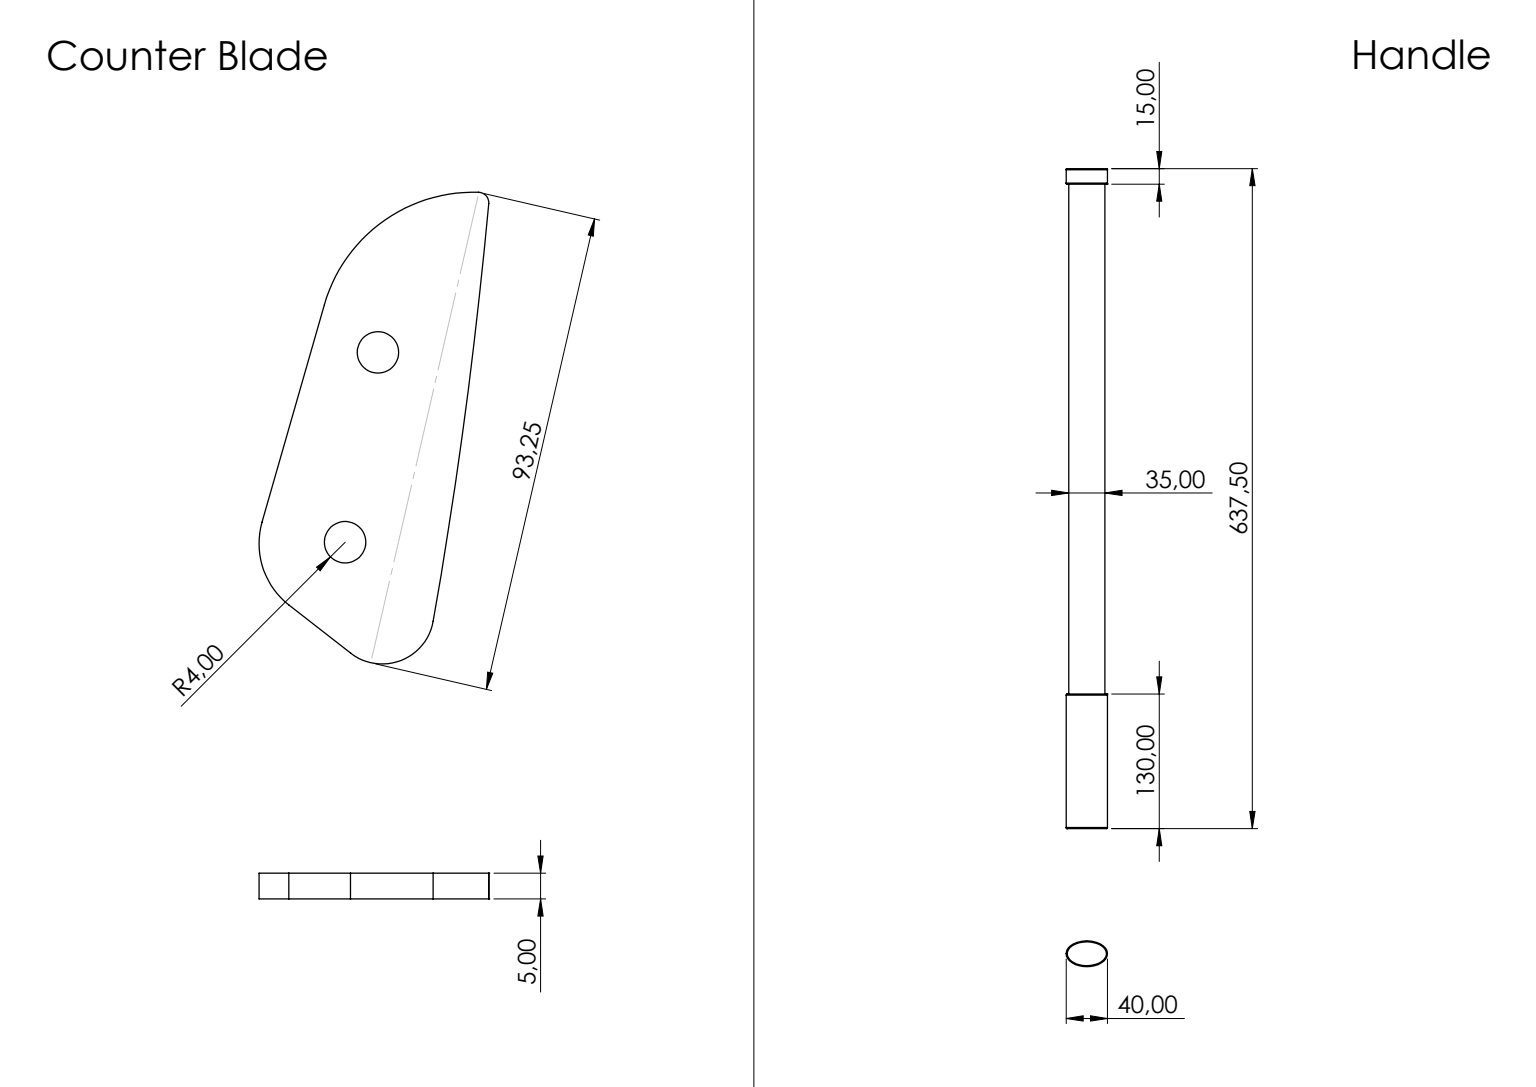
ISO-10303-21;
HEADER;
FILE_DESCRIPTION (('STEP AP214'),
    '1' );
FILE_NAME ('Counter Blade.step',
    '2026-10-06T08:24:18',
    ( '' ),
    ( '' ),
    'SwSTEP 2.0',
    'SolidWorks 2020',
    '' );
FILE_SCHEMA (( 'AUTOMOTIVE_DESIGN' ));
ENDSEC;

DATA;
#10=ORIENTED_EDGE ( 'NONE', *, *, #9690, .T. ) ;
#46=SHAPE_REPRESENTATION_RELATIONSHIP ( 'NONE' , 'NONE' ,  #1832, #4657 ) ;
#47=ADVANCED_FACE ( 'NONE', ( #10008 ), #1731, .T. ) ;
#57=AXIS2_PLACEMENT_3D ( 'NONE', #266, #1824, #2572 ) ;
#90=CARTESIAN_POINT ( 'NONE',  ( -6.594989095229207621, -2.500000000000000000, -526.5005977704149700 ) ) ;
#108=ORIENTED_EDGE ( 'NONE', *, *, #6819, .T. ) ;
#128=UNCERTAINTY_MEASURE_WITH_UNIT (LENGTH_MEASURE( 1.000000000000000082E-05 ), #4984, 'distance_accuracy_value', 'NONE');
#150=DIRECTION ( 'NONE',  ( 0.000000000000000000, 1.000000000000000000, -0.000000000000000000 ) ) ;
#154=LINE ( 'NONE', #4186, #6919 ) ;
#194=DIRECTION ( 'NONE',  ( 0.000000000000000000, 1.000000000000000000, -0.000000000000000000 ) ) ;
#199=VERTEX_POINT ( 'NONE', #5447 ) ;
#218=AXIS2_PLACEMENT_3D ( 'NONE', #4647, #8943, #6415 ) ;
#229=AXIS2_PLACEMENT_3D ( 'NONE', #4133, #4730, #3920 ) ;
#252=FACE_OUTER_BOUND ( 'NONE', #958, .T. ) ;
#266=CARTESIAN_POINT ( 'NONE',  ( -28.01838671672410896, -7.500000000000000000, -497.7560445212019999 ) ) ;
#274=CARTESIAN_POINT ( 'NONE',  ( -24.05731444175778577, -2.500000000000000000, -497.1993521173619683 ) ) ;
#286=PRODUCT_DEFINITION ( 'UNKNOWN', '', #449, #10550 ) ;
#328=FILL_AREA_STYLE_COLOUR ( '', #2300 ) ;
#356=EDGE_LOOP ( 'NONE', ( #3781, #10603 ) ) ;
#358=CYLINDRICAL_SURFACE ( 'NONE', #9948, 4.000000000000000000 ) ;
#380=DIRECTION ( 'NONE',  ( -0.9612616959383296633, 0.000000000000000000, -0.2756373558169616933 ) ) ;
#449=PRODUCT_DEFINITION_FORMATION_WITH_SPECIFIED_SOURCE ( 'ANY', '', #8602, .NOT_KNOWN. ) ;
#467=PRODUCT_DEFINITION_SHAPE ( 'NONE', 'NONE',  #286 ) ;
#471=VERTEX_POINT ( 'NONE', #3146 ) ;
#479=CARTESIAN_POINT ( 'NONE',  ( -30.41084982323499730, -2.500000000000000000, -460.5301199443746327 ) ) ;
#492=CARTESIAN_POINT ( 'NONE',  ( -36.01445213885307339, -7.500000000000000000, -460.8005622778243264 ) ) ;
#498=PLANE ( 'NONE',  #1895 ) ;
#557=AXIS2_PLACEMENT_3D ( 'NONE', #8920, #6558, #7364 ) ;
#585=DIRECTION ( 'NONE',  ( 0.000000000000000000, 1.000000000000000000, -0.000000000000000000 ) ) ;
#595=AXIS2_PLACEMENT_3D ( 'NONE', #9903, #3452, #2538 ) ;
#688=EDGE_LOOP ( 'NONE', ( #10453, #7051, #5685, #108 ) ) ;
#691=CARTESIAN_POINT ( 'NONE',  ( -1002.398135702230206, -7.500000000000000000, -618.0215964952759577 ) ) ;
#726=VERTEX_POINT ( 'NONE', #7376 ) ;
#745=DIRECTION ( 'NONE',  ( 0.000000000000000000, 1.000000000000000000, -0.000000000000000000 ) ) ;
#772=UNCERTAINTY_MEASURE_WITH_UNIT (LENGTH_MEASURE( 1.000000000000000082E-05 ), #971, 'distance_accuracy_value', 'NONE');
#788=ORIENTED_EDGE ( 'NONE', *, *, #10618, .F. ) ;
#791=ORIENTED_EDGE ( 'NONE', *, *, #4315, .T. ) ;
#819=ADVANCED_FACE ( 'NONE', ( #8387 ), #3450, .T. ) ;
#898=FILL_AREA_STYLE_COLOUR ( '', #2976 ) ;
#926=VECTOR ( 'NONE', #7594, 1000.000000000000227 ) ;
#927=ORIENTED_EDGE ( 'NONE', *, *, #1491, .T. ) ;
#933=CIRCLE ( 'NONE', #9689, 10.00000000000000178 ) ;
#958=EDGE_LOOP ( 'NONE', ( #5843, #3891, #8722, #3360 ) ) ;
#964=ADVANCED_FACE ( 'NONE', ( #9287 ), #358, .F. ) ;
#971=( LENGTH_UNIT ( ) NAMED_UNIT ( * ) SI_UNIT ( .MILLI., .METRE. ) );
#1064=ORIENTED_EDGE ( 'NONE', *, *, #5099, .F. ) ;
#1076=CIRCLE ( 'NONE', #229, 10.00000000000001599 ) ;
#1082=UNCERTAINTY_MEASURE_WITH_UNIT (LENGTH_MEASURE( 1.000000000000000082E-05 ), #1763, 'distance_accuracy_value', 'NONE');
#1091=CARTESIAN_POINT ( 'NONE',  ( -9.542482902900836450, -2.500000000000000000, -498.6999609700373526 ) ) ;
#1094=ADVANCED_FACE ( 'NONE', ( #9274 ), #5124, .T. ) ;
#1098=CIRCLE ( 'NONE', #1446, 4.000000000000000000 ) ;
#1129=PRESENTATION_STYLE_ASSIGNMENT (( #3395 ) ) ;
#1155=EDGE_LOOP ( 'NONE', ( #7696, #1064, #1796, #10507 ) ) ;
#1171=CARTESIAN_POINT ( 'NONE',  ( -38.33299437316763658, -7.500000000000000000, -461.6435047520546391 ) ) ;
#1209=DIRECTION ( 'NONE',  ( 0.000000000000000000, 1.000000000000000000, -0.000000000000000000 ) ) ;
#1225=DIRECTION ( 'NONE',  ( 0.000000000000000000, 1.000000000000000000, -0.000000000000000000 ) ) ;
#1279=DIRECTION ( 'NONE',  ( 0.000000000000000000, 1.000000000000000000, -0.000000000000000000 ) ) ;
#1282=AXIS2_PLACEMENT_3D ( 'NONE', #5388, #3631, #4388 ) ;
#1287=ADVANCED_FACE ( 'NONE', ( #1841, #7740, #3559 ), #8492, .T. ) ;
#1294=CARTESIAN_POINT ( 'NONE',  ( -50.43337757792475173, -7.500000000000000000, -464.9351226150769207 ) ) ;
#1402=DIRECTION ( 'NONE',  ( 0.000000000000000000, -1.000000000000000000, -0.000000000000000000 ) ) ;
#1416=VERTEX_POINT ( 'NONE', #7205 ) ;
#1428=DIRECTION ( 'NONE',  ( 0.000000000000000000, -1.000000000000000000, 0.000000000000000000 ) ) ;
#1446=AXIS2_PLACEMENT_3D ( 'NONE', #2951, #3606, #3652 ) ;
#1463=DIRECTION ( 'NONE',  ( 0.000000000000000000, 1.000000000000000000, -0.000000000000000000 ) ) ;
#1491=EDGE_CURVE ( 'NONE', #3141, #3262, #1508, .T. ) ;
#1492=FACE_OUTER_BOUND ( 'NONE', #688, .T. ) ;
#1508=LINE ( 'NONE', #8502, #7111 ) ;
#1544=DIRECTION ( 'NONE',  ( 0.9902680687415800209, 0.000000000000000000, 0.1391731009599966873 ) ) ;
#1552=( NAMED_UNIT ( * ) PLANE_ANGLE_UNIT ( ) SI_UNIT ( $, .RADIAN. ) );
#1553=EDGE_CURVE ( 'NONE', #471, #9652, #10117, .T. ) ;
#1577=EDGE_CURVE ( 'NONE', #3224, #9652, #4271, .T. ) ;
#1588=ORIENTED_EDGE ( 'NONE', *, *, #1491, .F. ) ;
#1602=CIRCLE ( 'NONE', #8454, 29.99999999999998224 ) ;
#1620=FACE_OUTER_BOUND ( 'NONE', #6632, .T. ) ;
#1669=CYLINDRICAL_SURFACE ( 'NONE', #557, 2.000000000000003997 ) ;
#1680=EDGE_LOOP ( 'NONE', ( #8671, #5541, #1588, #1899 ) ) ;
#1731=PLANE ( 'NONE',  #595 ) ;
#1763=( LENGTH_UNIT ( ) NAMED_UNIT ( * ) SI_UNIT ( .MILLI., .METRE. ) );
#1773=ORIENTED_EDGE ( 'NONE', *, *, #3982, .F. ) ;
#1781=CARTESIAN_POINT ( 'NONE',  ( -50.43337757792475173, -2.500000000000000000, -464.9351226150769207 ) ) ;
#1796=ORIENTED_EDGE ( 'NONE', *, *, #9999, .T. ) ;
#1824=DIRECTION ( 'NONE',  ( 0.000000000000000000, 1.000000000000000000, -0.000000000000000000 ) ) ;
#1832=SHAPE_REPRESENTATION ( 'Counter Blade', ( #2817 ), #5369 ) ;
#1841=FACE_BOUND ( 'NONE', #5066, .T. ) ;
#1889=SURFACE_SIDE_STYLE ('',( #10003 ) ) ;
#1895=AXIS2_PLACEMENT_3D ( 'NONE', #7059, #1402, #2107 ) ;
#1899=ORIENTED_EDGE ( 'NONE', *, *, #7170, .T. ) ;
#1905=ORIENTED_EDGE ( 'NONE', *, *, #4115, .F. ) ;
#1958=DIRECTION ( 'NONE',  ( -0.9902680687415801319, 0.000000000000000000, -0.1391731009599957991 ) ) ;
#1967=CARTESIAN_POINT ( 'NONE',  ( -38.33299437316763658, -7.500000000000000000, -461.6435047520546391 ) ) ;
#1999=DIRECTION ( 'NONE',  ( 0.000000000000000000, -1.000000000000000000, -0.000000000000000000 ) ) ;
#2026=CIRCLE ( 'NONE', #9059, 15.00000000000000533 ) ;
#2034=ORIENTED_EDGE ( 'NONE', *, *, #1553, .F. ) ;
#2039=CARTESIAN_POINT ( 'NONE',  ( -31.97945899169042505, -7.500000000000000000, -498.3127369250419747 ) ) ;
#2048=EDGE_CURVE ( 'NONE', #3465, #199, #5327, .T. ) ;
#2051=CARTESIAN_POINT ( 'NONE',  ( -38.38033378105252780, -7.500000000000000000, -506.9690816445435644 ) ) ;
#2055=CARTESIAN_POINT ( 'NONE',  ( -8.586595388443328147, -7.500000000000000000, -526.6836397678595176 ) ) ;
#2065=DIRECTION ( 'NONE',  ( 0.000000000000000000, -1.000000000000000000, 0.000000000000000000 ) ) ;
#2107=DIRECTION ( 'NONE',  ( -0.9902680687415799099, 0.000000000000000000, -0.1391731009599969648 ) ) ;
#2116=CARTESIAN_POINT ( 'NONE',  ( -38.38033378105252780, -2.500000000000000000, -506.9690816445435644 ) ) ;
#2145=CARTESIAN_POINT ( 'NONE',  ( -8.518317708839887814, -7.500000000000000000, -528.6824739677025491 ) ) ;
#2214=DIRECTION ( 'NONE',  ( 0.9902680687415800209, 0.000000000000000000, 0.1391731009599966873 ) ) ;
#2245=DIRECTION ( 'NONE',  ( 0.9958031466069998672, 0.000000000000000000, 0.09152099872487109988 ) ) ;
#2264=EDGE_CURVE ( 'NONE', #3224, #3141, #2026, .T. ) ;
#2266=LINE ( 'NONE', #5533, #6349 ) ;
#2291=VECTOR ( 'NONE', #585, 1000.000000000000000 ) ;
#2300=COLOUR_RGB ( '', 0.09019608, 0.27058824, 0.51372549) ;
#2318=DIRECTION ( 'NONE',  ( 0.000000000000000000, 1.000000000000000000, -0.000000000000000000 ) ) ;
#2325=ORIENTED_EDGE ( 'NONE', *, *, #2474, .F. ) ;
#2336=ORIENTED_EDGE ( 'NONE', *, *, #1553, .T. ) ;
#2372=LINE ( 'NONE', #7314, #10423 ) ;
#2373=CARTESIAN_POINT ( 'NONE',  ( -34.37192209820132405, -7.500000000000000000, -461.0868123482146643 ) ) ;
#2408=CARTESIAN_POINT ( 'NONE',  ( -50.43337757792475173, -7.500000000000000000, -464.9351226150769207 ) ) ;
#2409=AXIS2_PLACEMENT_3D ( 'NONE', #10577, #745, #5681 ) ;
#2445=FACE_OUTER_BOUND ( 'NONE', #1155, .T. ) ;
#2446=ORIENTED_EDGE ( 'NONE', *, *, #3484, .T. ) ;
#2457=VECTOR ( 'NONE', #2065, 1000.000000000000000 ) ;
#2474=EDGE_CURVE ( 'NONE', #7593, #3224, #2372, .T. ) ;
#2495=CARTESIAN_POINT ( 'NONE',  ( -34.37192209820132405, -7.500000000000000000, -461.0868123482146643 ) ) ;
#2511=DIRECTION ( 'NONE',  ( 0.000000000000000000, 1.000000000000000000, -0.000000000000000000 ) ) ;
#2538=DIRECTION ( 'NONE',  ( 0.000000000000000000, 1.000000000000000000, -0.000000000000000000 ) ) ;
#2550=CYLINDRICAL_SURFACE ( 'NONE', #7930, 10.00000000000001599 ) ;
#2572=DIRECTION ( 'NONE',  ( -0.9902680687415800209, 0.000000000000000000, -0.1391731009599967983 ) ) ;
#2623=DIRECTION ( 'NONE',  ( 0.9902680687415800209, 0.000000000000000000, 0.1391731009599966873 ) ) ;
#2659=ORIENTED_EDGE ( 'NONE', *, *, #6694, .F. ) ;
#2661=EDGE_LOOP ( 'NONE', ( #3907, #10072, #9299, #3463 ) ) ;
#2702=CARTESIAN_POINT ( 'NONE',  ( -19.08872200864999868, -7.500000000000000000, -429.3350920981999934 ) ) ;
#2709=DIRECTION ( 'NONE',  ( 0.03413883980201725538, 0.000000000000000000, -0.9994170999222358187 ) ) ;
#2757=CIRCLE ( 'NONE', #6859, 999.9999999999997726 ) ;
#2758=CARTESIAN_POINT ( 'NONE',  ( -33.34106825788445150, -2.500000000000000000, -439.6766126514281154 ) ) ;
#2767=FACE_BOUND ( 'NONE', #4216, .T. ) ;
#2817=AXIS2_PLACEMENT_3D ( 'NONE', #8634, #3966, #3161 ) ;
#2835=CIRCLE ( 'NONE', #1282, 29.99999999999998224 ) ;
#2951=CARTESIAN_POINT ( 'NONE',  ( -28.01838671672410896, -7.500000000000000000, -497.7560445212019999 ) ) ;
#2976=COLOUR_RGB ( '', 0.09019608, 0.27058824, 0.51372549) ;
#2997=AXIS2_PLACEMENT_3D ( 'NONE', #7933, #9712, #1544 ) ;
#3058=ORIENTED_EDGE ( 'NONE', *, *, #7135, .T. ) ;
#3127=ORIENTED_EDGE ( 'NONE', *, *, #6034, .T. ) ;
#3131=EDGE_LOOP ( 'NONE', ( #791, #3679 ) ) ;
#3138=DIRECTION ( 'NONE',  ( -0.9612616959383299964, 0.000000000000000000, -0.2756373558169601945 ) ) ;
#3141=VERTEX_POINT ( 'NONE', #1294 ) ;
#3142=FACE_OUTER_BOUND ( 'NONE', #9330, .T. ) ;
#3146=CARTESIAN_POINT ( 'NONE',  ( -33.34106825788445150, -2.500000000000000000, -439.6766126514281154 ) ) ;
#3150=CIRCLE ( 'NONE', #9164, 14.99999999999999112 ) ;
#3157=CARTESIAN_POINT ( 'NONE',  ( -8.518317708839887814, -2.500000000000000000, -528.6824739677025491 ) ) ;
#3158=CARTESIAN_POINT ( 'NONE',  ( -8.586595388443328147, -2.500000000000000000, -526.6836397678595176 ) ) ;
#3161=DIRECTION ( 'NONE',  ( 1.000000000000000000, 0.000000000000000000, 0.000000000000000000 ) ) ;
#3209=EDGE_LOOP ( 'NONE', ( #3058, #3445, #4855, #6669, #927, #4767, #7906 ) ) ;
#3224=VERTEX_POINT ( 'NONE', #7055 ) ;
#3228=FACE_OUTER_BOUND ( 'NONE', #3258, .T. ) ;
#3258=EDGE_LOOP ( 'NONE', ( #5813, #4124, #3127, #7270 ) ) ;
#3262=VERTEX_POINT ( 'NONE', #2051 ) ;
#3329=ORIENTED_EDGE ( 'NONE', *, *, #8250, .F. ) ;
#3351=ADVANCED_FACE ( 'NONE', ( #3228 ), #8062, .F. ) ;
#3360=ORIENTED_EDGE ( 'NONE', *, *, #8250, .T. ) ;
#3379=ADVANCED_FACE ( 'NONE', ( #1620 ), #1669, .T. ) ;
#3395=SURFACE_STYLE_USAGE ( .BOTH. , #1889 ) ;
#3424=CARTESIAN_POINT ( 'NONE',  ( -34.37192209820132405, -7.500000000000000000, -461.0868123482146643 ) ) ;
#3439=AXIS2_PLACEMENT_3D ( 'NONE', #7852, #10078, #2214 ) ;
#3445=ORIENTED_EDGE ( 'NONE', *, *, #5099, .T. ) ;
#3450=PLANE ( 'NONE',  #5140 ) ;
#3452=DIRECTION ( 'NONE',  ( -0.6156614753245244209, 0.000000000000000000, 0.7880107536076078611 ) ) ;
#3463=ORIENTED_EDGE ( 'NONE', *, *, #10535, .F. ) ;
#3464=DIRECTION ( 'NONE',  ( 0.000000000000000000, 1.000000000000000000, -0.000000000000000000 ) ) ;
#3465=VERTEX_POINT ( 'NONE', #2039 ) ;
#3484=EDGE_CURVE ( 'NONE', #7857, #199, #8968, .T. ) ;
#3505=CARTESIAN_POINT ( 'NONE',  ( -53.22217373880035041, -2.500000000000000000, -455.2094346026838139 ) ) ;
#3529=ORIENTED_EDGE ( 'NONE', *, *, #8365, .F. ) ;
#3546=EDGE_LOOP ( 'NONE', ( #1905, #1773, #10, #788 ) ) ;
#3559=FACE_OUTER_BOUND ( 'NONE', #3209, .T. ) ;
#3606=DIRECTION ( 'NONE',  ( 0.000000000000000000, 1.000000000000000000, -0.000000000000000000 ) ) ;
#3626=CARTESIAN_POINT ( 'NONE',  ( -36.01445213885307339, -7.656480000000000175, -460.8005622778243264 ) ) ;
#3631=DIRECTION ( 'NONE',  ( 0.000000000000000000, -1.000000000000000000, 0.000000000000000000 ) ) ;
#3636=CARTESIAN_POINT ( 'NONE',  ( -28.01838671672410896, -7.500000000000000000, -497.7560445212019999 ) ) ;
#3641=VECTOR ( 'NONE', #4192, 1000.000000000000227 ) ;
#3652=DIRECTION ( 'NONE',  ( 0.9902680687415800209, 0.000000000000000000, 0.1391731009599966873 ) ) ;
#3679=ORIENTED_EDGE ( 'NONE', *, *, #8962, .T. ) ;
#3710=EDGE_CURVE ( 'NONE', #7593, #471, #154, .T. ) ;
#3768=DIRECTION ( 'NONE',  ( 0.000000000000000000, 1.000000000000000000, -0.000000000000000000 ) ) ;
#3781=ORIENTED_EDGE ( 'NONE', *, *, #6819, .F. ) ;
#3881=CYLINDRICAL_SURFACE ( 'NONE', #3439, 4.000000000000000000 ) ;
#3891=ORIENTED_EDGE ( 'NONE', *, *, #7244, .F. ) ;
#3907=ORIENTED_EDGE ( 'NONE', *, *, #7170, .F. ) ;
#3920=DIRECTION ( 'NONE',  ( -0.6156614753245235327, 0.000000000000000000, 0.7880107536076085273 ) ) ;
#3944=CARTESIAN_POINT ( 'NONE',  ( -9.542482902900836450, -7.500000000000000000, -498.6999609700373526 ) ) ;
#3966=DIRECTION ( 'NONE',  ( 0.000000000000000000, 0.000000000000000000, 1.000000000000000000 ) ) ;
#3976=VECTOR ( 'NONE', #5351, 1000.000000000000000 ) ;
#3982=EDGE_CURVE ( 'NONE', #9423, #3262, #8509, .T. ) ;
#4038=SHAPE_DEFINITION_REPRESENTATION ( #467, #1832 ) ;
#4076=( NAMED_UNIT ( * ) SI_UNIT ( $, .STERADIAN. ) SOLID_ANGLE_UNIT ( ) );
#4115=EDGE_CURVE ( 'NONE', #3262, #7113, #1602, .T. ) ;
#4124=ORIENTED_EDGE ( 'NONE', *, *, #7586, .F. ) ;
#4130=AXIS2_PLACEMENT_3D ( 'NONE', #8785, #1428, #4714 ) ;
#4133=CARTESIAN_POINT ( 'NONE',  ( -27.18445350464674348, -2.500000000000000000, -447.5567201875090291 ) ) ;
#4186=CARTESIAN_POINT ( 'NONE',  ( -33.34106825788445150, -7.500000000000000000, -439.6766126514281154 ) ) ;
#4192=DIRECTION ( 'NONE',  ( 0.2756373558169616378, 0.000000000000000000, -0.9612616959383295523 ) ) ;
#4216=EDGE_LOOP ( 'NONE', ( #2659, #3329 ) ) ;
#4221=LINE ( 'NONE', #8295, #5908 ) ;
#4257=( NAMED_UNIT ( * ) PLANE_ANGLE_UNIT ( ) SI_UNIT ( $, .RADIAN. ) );
#4259=EDGE_CURVE ( 'NONE', #471, #6686, #1076, .T. ) ;
#4271=LINE ( 'NONE', #7541, #8819 ) ;
#4303=AXIS2_PLACEMENT_3D ( 'NONE', #3158, #8905, #8793 ) ;
#4315=EDGE_CURVE ( 'NONE', #3465, #8821, #8795, .T. ) ;
#4388=DIRECTION ( 'NONE',  ( -0.9612616959383299964, 0.000000000000000000, -0.2756373558169601945 ) ) ;
#4440=DIRECTION ( 'NONE',  ( 0.9902680687415800209, 0.000000000000000000, 0.1391731009599966873 ) ) ;
#4499=DIRECTION ( 'NONE',  ( -0.9902680687415800209, 0.000000000000000000, -0.1391731009599967983 ) ) ;
#4647=CARTESIAN_POINT ( 'NONE',  ( -1002.398135702230206, -2.500000000000000000, -618.0215964952759577 ) ) ;
#4657=ADVANCED_BREP_SHAPE_REPRESENTATION ( '', ( #8917, #2817 ), #5369 ) ;
#4694=ADVANCED_FACE ( 'NONE', ( #9005 ), #6691, .T. ) ;
#4714=DIRECTION ( 'NONE',  ( 0.9958031466069998672, 0.000000000000000000, 0.09152099872487109988 ) ) ;
#4727=LINE ( 'NONE', #2145, #2291 ) ;
#4730=DIRECTION ( 'NONE',  ( 0.000000000000000000, 1.000000000000000000, -0.000000000000000000 ) ) ;
#4767=ORIENTED_EDGE ( 'NONE', *, *, #4115, .T. ) ;
#4791=EDGE_CURVE ( 'NONE', #8821, #7857, #4221, .T. ) ;
#4845=CARTESIAN_POINT ( 'NONE',  ( -24.05731444175778577, -7.500000000000000000, -497.1993521173619683 ) ) ;
#4855=ORIENTED_EDGE ( 'NONE', *, *, #2474, .T. ) ;
#4882=( NAMED_UNIT ( * ) PLANE_ANGLE_UNIT ( ) SI_UNIT ( $, .RADIAN. ) );
#4984=( LENGTH_UNIT ( ) NAMED_UNIT ( * ) SI_UNIT ( .MILLI., .METRE. ) );
#5032=MECHANICAL_DESIGN_GEOMETRIC_PRESENTATION_REPRESENTATION('',(#5209),#7957);
#5066=EDGE_LOOP ( 'NONE', ( #8248, #8698 ) ) ;
#5078=LINE ( 'NONE', #5944, #9694 ) ;
#5094=ORIENTED_EDGE ( 'NONE', *, *, #7000, .T. ) ;
#5099=EDGE_CURVE ( 'NONE', #1416, #7593, #933, .T. ) ;
#5124=CYLINDRICAL_SURFACE ( 'NONE', #6944, 29.99999999999999289 ) ;
#5140=AXIS2_PLACEMENT_3D ( 'NONE', #3505, #380, #8335 ) ;
#5209=STYLED_ITEM ( 'NONE', ( #8160 ), #4657 ) ;
#5235=ORIENTED_EDGE ( 'NONE', *, *, #7135, .F. ) ;
#5241=ORIENTED_EDGE ( 'NONE', *, *, #4259, .T. ) ;
#5255=SURFACE_SIDE_STYLE ('',( #8316 ) ) ;
#5306=CARTESIAN_POINT ( 'NONE',  ( -28.01838671672410896, -2.500000000000000000, -497.7560445212019999 ) ) ;
#5327=LINE ( 'NONE', #6190, #7681 ) ;
#5350=VERTEX_POINT ( 'NONE', #1967 ) ;
#5351=DIRECTION ( 'NONE',  ( 0.000000000000000000, 1.000000000000000000, -0.000000000000000000 ) ) ;
#5369=( GEOMETRIC_REPRESENTATION_CONTEXT ( 3 ) GLOBAL_UNCERTAINTY_ASSIGNED_CONTEXT ( ( #128 ) ) GLOBAL_UNIT_ASSIGNED_CONTEXT ( ( #4984, #4882, #5733 ) ) REPRESENTATION_CONTEXT ( 'NONE', 'WORKASPACE' ) );
#5382=CLOSED_SHELL ( 'NONE', ( #3351, #8609, #9379, #964, #1287, #6194, #6341, #47, #4694, #819, #1094, #3379, #8631 ) ) ;
#5388=CARTESIAN_POINT ( 'NONE',  ( -9.542482902900836450, -2.500000000000000000, -498.6999609700373526 ) ) ;
#5422=DIRECTION ( 'NONE',  ( -0.6156614753245245319, 0.000000000000000000, 0.7880107536076076391 ) ) ;
#5423=AXIS2_PLACEMENT_3D ( 'NONE', #2702, #1999, #7533 ) ;
#5447=CARTESIAN_POINT ( 'NONE',  ( -31.97945899169042505, -2.500000000000000000, -498.3127369250419747 ) ) ;
#5457=LINE ( 'NONE', #1171, #3976 ) ;
#5463=CARTESIAN_POINT ( 'NONE',  ( -36.01445213885307339, -2.500000000000000000, -460.8005622778243264 ) ) ;
#5533=CARTESIAN_POINT ( 'NONE',  ( -30.41084982323499730, -7.500000000000000000, -460.5301199443746327 ) ) ;
#5541=ORIENTED_EDGE ( 'NONE', *, *, #3982, .T. ) ;
#5579=CARTESIAN_POINT ( 'NONE',  ( -38.33299437316763658, -2.500000000000000000, -461.6435047520546391 ) ) ;
#5648=AXIS2_PLACEMENT_3D ( 'NONE', #3424, #150, #2623 ) ;
#5681=DIRECTION ( 'NONE',  ( 0.9902680687415800209, 0.000000000000000000, 0.1391731009599966873 ) ) ;
#5685=ORIENTED_EDGE ( 'NONE', *, *, #2048, .T. ) ;
#5733=( NAMED_UNIT ( * ) SI_UNIT ( $, .STERADIAN. ) SOLID_ANGLE_UNIT ( ) );
#5741=CIRCLE ( 'NONE', #6247, 2.000000000000007550 ) ;
#5765=ORIENTED_EDGE ( 'NONE', *, *, #7000, .F. ) ;
#5813=ORIENTED_EDGE ( 'NONE', *, *, #8719, .F. ) ;
#5823=CIRCLE ( 'NONE', #4130, 999.9999999999997726 ) ;
#5837=FILL_AREA_STYLE ('',( #898 ) ) ;
#5843=ORIENTED_EDGE ( 'NONE', *, *, #6034, .F. ) ;
#5900=EDGE_CURVE ( 'NONE', #8899, #9423, #9938, .T. ) ;
#5908=VECTOR ( 'NONE', #194, 1000.000000000000000 ) ;
#5944=CARTESIAN_POINT ( 'NONE',  ( -6.594989095229207621, -7.500000000000000000, -526.5005977704149700 ) ) ;
#6034=EDGE_CURVE ( 'NONE', #5350, #9268, #5457, .T. ) ;
#6049=AXIS2_PLACEMENT_3D ( 'NONE', #5306, #1225, #9452 ) ;
#6098=ORIENTED_EDGE ( 'NONE', *, *, #2048, .F. ) ;
#6190=CARTESIAN_POINT ( 'NONE',  ( -31.97945899169042505, -7.500000000000000000, -498.3127369250419747 ) ) ;
#6194=ADVANCED_FACE ( 'NONE', ( #3142 ), #8837, .T. ) ;
#6247=AXIS2_PLACEMENT_3D ( 'NONE', #2055, #8595, #2709 ) ;
#6268=ORIENTED_EDGE ( 'NONE', *, *, #9945, .F. ) ;
#6341=ADVANCED_FACE ( 'NONE', ( #2445 ), #2550, .T. ) ;
#6349=VECTOR ( 'NONE', #1463, 1000.000000000000000 ) ;
#6370=ORIENTED_EDGE ( 'NONE', *, *, #9690, .F. ) ;
#6415=DIRECTION ( 'NONE',  ( -0.9902680687415799099, 0.000000000000000000, -0.1391731009599970204 ) ) ;
#6433=DIRECTION ( 'NONE',  ( 0.000000000000000000, 1.000000000000000000, -0.000000000000000000 ) ) ;
#6441=DIRECTION ( 'NONE',  ( 0.000000000000000000, -1.000000000000000000, 0.000000000000000000 ) ) ;
#6451=PRODUCT_CONTEXT ( 'NONE', #9844, 'mechanical' ) ;
#6516=CIRCLE ( 'NONE', #9431, 4.000000000000003553 ) ;
#6525=ORIENTED_EDGE ( 'NONE', *, *, #5900, .F. ) ;
#6539=CYLINDRICAL_SURFACE ( 'NONE', #2997, 4.000000000000000000 ) ;
#6558=DIRECTION ( 'NONE',  ( 0.000000000000000000, 1.000000000000000000, -0.000000000000000000 ) ) ;
#6624=CARTESIAN_POINT ( 'NONE',  ( -17.33381025012258903, -2.500000000000000000, -445.8348527500487535 ) ) ;
#6632=EDGE_LOOP ( 'NONE', ( #8804, #6268, #7935, #5765 ) ) ;
#6669=ORIENTED_EDGE ( 'NONE', *, *, #2264, .T. ) ;
#6686=VERTEX_POINT ( 'NONE', #6624 ) ;
#6691=CYLINDRICAL_SURFACE ( 'NONE', #8313, 14.99999999999999112 ) ;
#6694=EDGE_CURVE ( 'NONE', #9268, #10547, #9289, .T. ) ;
#6744=DIRECTION ( 'NONE',  ( 0.2756373558169616378, 0.000000000000000000, -0.9612616959383295523 ) ) ;
#6783=ORIENTED_EDGE ( 'NONE', *, *, #8962, .F. ) ;
#6819=EDGE_CURVE ( 'NONE', #199, #7857, #8932, .T. ) ;
#6859=AXIS2_PLACEMENT_3D ( 'NONE', #691, #8961, #2245 ) ;
#6908=DIRECTION ( 'NONE',  ( 0.000000000000000000, 1.000000000000000000, -0.000000000000000000 ) ) ;
#6919=VECTOR ( 'NONE', #8470, 1000.000000000000000 ) ;
#6944=AXIS2_PLACEMENT_3D ( 'NONE', #1091, #10073, #1958 ) ;
#6947=MECHANICAL_DESIGN_GEOMETRIC_PRESENTATION_REPRESENTATION('',(#8299),#9675);
#7000=EDGE_CURVE ( 'NONE', #8559, #10046, #7895, .T. ) ;
#7019=ORIENTED_EDGE ( 'NONE', *, *, #1577, .F. ) ;
#7037=CIRCLE ( 'NONE', #5648, 4.000000000000000000 ) ;
#7051=ORIENTED_EDGE ( 'NONE', *, *, #4315, .F. ) ;
#7055=CARTESIAN_POINT ( 'NONE',  ( -45.24937426871918689, -7.500000000000000000, -448.9804009737068213 ) ) ;
#7059=CARTESIAN_POINT ( 'NONE',  ( -19.08872200864999868, -2.500000000000000000, -429.3350920981999934 ) ) ;
#7111=VECTOR ( 'NONE', #6744, 1000.000000000000227 ) ;
#7113=VERTEX_POINT ( 'NONE', #9019 ) ;
#7135=EDGE_CURVE ( 'NONE', #8191, #1416, #2757, .T. ) ;
#7158=FACE_OUTER_BOUND ( 'NONE', #9944, .T. ) ;
#7170=EDGE_CURVE ( 'NONE', #3141, #8899, #9770, .T. ) ;
#7205=CARTESIAN_POINT ( 'NONE',  ( -17.33381025012258903, -7.500000000000000000, -445.8348527500487535 ) ) ;
#7244=EDGE_CURVE ( 'NONE', #726, #5350, #7037, .T. ) ;
#7270=ORIENTED_EDGE ( 'NONE', *, *, #6694, .T. ) ;
#7278=DIRECTION ( 'NONE',  ( 0.000000000000000000, -1.000000000000000000, 0.000000000000000000 ) ) ;
#7314=CARTESIAN_POINT ( 'NONE',  ( -33.34106825788445150, -7.500000000000000000, -439.6766126514281154 ) ) ;
#7363=DIRECTION ( 'NONE',  ( -0.7880107536076077501, 0.000000000000000000, -0.6156614753245244209 ) ) ;
#7364=DIRECTION ( 'NONE',  ( 0.9958031466069979798, 0.000000000000000000, 0.09152099872489198595 ) ) ;
#7367=AXIS2_PLACEMENT_3D ( 'NONE', #10357, #9500, #4499 ) ;
#7376=CARTESIAN_POINT ( 'NONE',  ( -30.41084982323499730, -7.500000000000000000, -460.5301199443746327 ) ) ;
#7460=SURFACE_STYLE_USAGE ( .BOTH. , #5255 ) ;
#7533=DIRECTION ( 'NONE',  ( -0.9902680687415799099, 0.000000000000000000, -0.1391731009599969648 ) ) ;
#7541=CARTESIAN_POINT ( 'NONE',  ( -45.24937426871918689, -7.500000000000000000, -448.9804009737068213 ) ) ;
#7543=CARTESIAN_POINT ( 'NONE',  ( -27.18445350464674348, -7.656480000000000175, -447.5567201875090291 ) ) ;
#7586=EDGE_CURVE ( 'NONE', #5350, #726, #6516, .T. ) ;
#7593=VERTEX_POINT ( 'NONE', #10066 ) ;
#7594=DIRECTION ( 'NONE',  ( -0.7880107536076077501, 0.000000000000000000, -0.6156614753245244209 ) ) ;
#7681=VECTOR ( 'NONE', #10384, 1000.000000000000000 ) ;
#7685=( NAMED_UNIT ( * ) SI_UNIT ( $, .STERADIAN. ) SOLID_ANGLE_UNIT ( ) );
#7696=ORIENTED_EDGE ( 'NONE', *, *, #3710, .F. ) ;
#7713=ORIENTED_EDGE ( 'NONE', *, *, #9542, .T. ) ;
#7727=ORIENTED_EDGE ( 'NONE', *, *, #10535, .T. ) ;
#7740=FACE_BOUND ( 'NONE', #3131, .T. ) ;
#7798=CARTESIAN_POINT ( 'NONE',  ( -17.33381025012248600, -7.500000000000000000, -445.8348527500487535 ) ) ;
#7852=CARTESIAN_POINT ( 'NONE',  ( -34.37192209820132405, -7.500000000000000000, -461.0868123482146643 ) ) ;
#7857=VERTEX_POINT ( 'NONE', #274 ) ;
#7895=CIRCLE ( 'NONE', #4303, 2.000000000000001776 ) ;
#7906=ORIENTED_EDGE ( 'NONE', *, *, #9945, .T. ) ;
#7930=AXIS2_PLACEMENT_3D ( 'NONE', #7543, #3464, #9109 ) ;
#7933=CARTESIAN_POINT ( 'NONE',  ( -28.01838671672410896, -7.500000000000000000, -497.7560445212019999 ) ) ;
#7935=ORIENTED_EDGE ( 'NONE', *, *, #10618, .T. ) ;
#7947=CARTESIAN_POINT ( 'NONE',  ( -27.18445350464674348, -7.500000000000000000, -447.5567201875090291 ) ) ;
#7955=DIRECTION ( 'NONE',  ( 0.000000000000000000, -1.000000000000000000, 0.000000000000000000 ) ) ;
#7957=( GEOMETRIC_REPRESENTATION_CONTEXT ( 3 ) GLOBAL_UNCERTAINTY_ASSIGNED_CONTEXT ( ( #1082 ) ) GLOBAL_UNIT_ASSIGNED_CONTEXT ( ( #1763, #1552, #4076 ) ) REPRESENTATION_CONTEXT ( 'NONE', 'WORKASPACE' ) );
#8062=CYLINDRICAL_SURFACE ( 'NONE', #9655, 4.000000000000000000 ) ;
#8160=PRESENTATION_STYLE_ASSIGNMENT (( #7460 ) ) ;
#8179=DIRECTION ( 'NONE',  ( -0.9902680687415800209, 0.000000000000000000, -0.1391731009599965763 ) ) ;
#8191=VERTEX_POINT ( 'NONE', #8743 ) ;
#8226=CARTESIAN_POINT ( 'NONE',  ( -34.37192209820132405, -2.500000000000000000, -461.0868123482146643 ) ) ;
#8245=VECTOR ( 'NONE', #6433, 1000.000000000000000 ) ;
#8248=ORIENTED_EDGE ( 'NONE', *, *, #7586, .T. ) ;
#8250=EDGE_CURVE ( 'NONE', #10547, #9268, #9785, .T. ) ;
#8289=EDGE_LOOP ( 'NONE', ( #2325, #9089, #2336, #7019 ) ) ;
#8295=CARTESIAN_POINT ( 'NONE',  ( -24.05731444175778577, -7.500000000000000000, -497.1993521173619683 ) ) ;
#8299=STYLED_ITEM ( 'NONE', ( #1129 ), #8917 ) ;
#8313=AXIS2_PLACEMENT_3D ( 'NONE', #3626, #6908, #9970 ) ;
#8316=SURFACE_STYLE_FILL_AREA ( #5837 ) ;
#8323=ORIENTED_EDGE ( 'NONE', *, *, #8365, .T. ) ;
#8335=DIRECTION ( 'NONE',  ( 0.000000000000000000, 1.000000000000000000, -0.000000000000000000 ) ) ;
#8347=EDGE_LOOP ( 'NONE', ( #6098, #6783, #8828, #2446 ) ) ;
#8365=EDGE_CURVE ( 'NONE', #8559, #6686, #5823, .T. ) ;
#8375=CARTESIAN_POINT ( 'NONE',  ( -50.43337757792475173, -2.500000000000000000, -464.9351226150769207 ) ) ;
#8387=FACE_OUTER_BOUND ( 'NONE', #1680, .T. ) ;
#8396=LINE ( 'NONE', #7798, #9868 ) ;
#8454=AXIS2_PLACEMENT_3D ( 'NONE', #3944, #7278, #3138 ) ;
#8470=DIRECTION ( 'NONE',  ( 0.000000000000000000, 1.000000000000000000, -0.000000000000000000 ) ) ;
#8492=PLANE ( 'NONE',  #5423 ) ;
#8502=CARTESIAN_POINT ( 'NONE',  ( -50.43337757792475173, -7.500000000000000000, -464.9351226150769207 ) ) ;
#8509=LINE ( 'NONE', #2116, #2457 ) ;
#8559=VERTEX_POINT ( 'NONE', #90 ) ;
#8595=DIRECTION ( 'NONE',  ( 0.000000000000000000, -1.000000000000000000, 0.000000000000000000 ) ) ;
#8602=PRODUCT ( 'Counter Blade', 'Counter Blade', '', ( #6451 ) ) ;
#8609=ADVANCED_FACE ( 'NONE', ( #252 ), #3881, .F. ) ;
#8631=ADVANCED_FACE ( 'NONE', ( #2767, #9466, #7158 ), #498, .F. ) ;
#8634=CARTESIAN_POINT ( 'NONE',  ( 0.000000000000000000, 0.000000000000000000, 0.000000000000000000 ) ) ;
#8671=ORIENTED_EDGE ( 'NONE', *, *, #5900, .T. ) ;
#8698=ORIENTED_EDGE ( 'NONE', *, *, #7244, .T. ) ;
#8719=EDGE_CURVE ( 'NONE', #726, #10547, #2266, .T. ) ;
#8722=ORIENTED_EDGE ( 'NONE', *, *, #8719, .T. ) ;
#8743=CARTESIAN_POINT ( 'NONE',  ( -6.594989095229207621, -7.500000000000000000, -526.5005977704149700 ) ) ;
#8785=CARTESIAN_POINT ( 'NONE',  ( -1002.398135702230206, -2.500000000000000000, -618.0215964952759577 ) ) ;
#8793=DIRECTION ( 'NONE',  ( 0.9958031466069877657, 0.000000000000000000, 0.09152099872500310540 ) ) ;
#8795=CIRCLE ( 'NONE', #57, 3.999999999999996447 ) ;
#8804=ORIENTED_EDGE ( 'NONE', *, *, #9542, .F. ) ;
#8819=VECTOR ( 'NONE', #3768, 1000.000000000000000 ) ;
#8821=VERTEX_POINT ( 'NONE', #4845 ) ;
#8828=ORIENTED_EDGE ( 'NONE', *, *, #4791, .T. ) ;
#8837=CYLINDRICAL_SURFACE ( 'NONE', #218, 1000.000000000000000 ) ;
#8850=CARTESIAN_POINT ( 'NONE',  ( -38.38033378105252780, -2.500000000000000000, -506.9690816445435644 ) ) ;
#8899=VERTEX_POINT ( 'NONE', #1781 ) ;
#8902=ORIENTED_EDGE ( 'NONE', *, *, #9999, .F. ) ;
#8905=DIRECTION ( 'NONE',  ( 0.000000000000000000, 1.000000000000000000, -0.000000000000000000 ) ) ;
#8917=MANIFOLD_SOLID_BREP ( 'Stock-MAS-686-1', #5382 ) ;
#8920=CARTESIAN_POINT ( 'NONE',  ( -8.586595388443328147, -7.656480000000000175, -526.6836397678595176 ) ) ;
#8932=CIRCLE ( 'NONE', #7367, 3.999999999999996447 ) ;
#8943=DIRECTION ( 'NONE',  ( 0.000000000000000000, -1.000000000000000000, 0.000000000000000000 ) ) ;
#8961=DIRECTION ( 'NONE',  ( 0.000000000000000000, -1.000000000000000000, 0.000000000000000000 ) ) ;
#8962=EDGE_CURVE ( 'NONE', #8821, #3465, #1098, .T. ) ;
#8968=CIRCLE ( 'NONE', #6049, 4.000000000000000000 ) ;
#9005=FACE_OUTER_BOUND ( 'NONE', #2661, .T. ) ;
#9019=CARTESIAN_POINT ( 'NONE',  ( -8.518317708839887814, -7.500000000000000000, -528.6824739677025491 ) ) ;
#9059=AXIS2_PLACEMENT_3D ( 'NONE', #492, #7955, #5422 ) ;
#9089=ORIENTED_EDGE ( 'NONE', *, *, #3710, .T. ) ;
#9109=DIRECTION ( 'NONE',  ( -0.6156614753245235327, 0.000000000000000000, 0.7880107536076085273 ) ) ;
#9154=DIRECTION ( 'NONE',  ( 0.000000000000000000, 1.000000000000000000, -0.000000000000000000 ) ) ;
#9164=AXIS2_PLACEMENT_3D ( 'NONE', #5463, #1279, #9504 ) ;
#9258=FILL_AREA_STYLE ('',( #328 ) ) ;
#9268=VERTEX_POINT ( 'NONE', #5579 ) ;
#9274=FACE_OUTER_BOUND ( 'NONE', #3546, .T. ) ;
#9287=FACE_OUTER_BOUND ( 'NONE', #8347, .T. ) ;
#9289=CIRCLE ( 'NONE', #10137, 4.000000000000003553 ) ;
#9299=ORIENTED_EDGE ( 'NONE', *, *, #1577, .T. ) ;
#9330=EDGE_LOOP ( 'NONE', ( #8323, #8902, #5235, #7713 ) ) ;
#9379=ADVANCED_FACE ( 'NONE', ( #1492 ), #6539, .F. ) ;
#9420=DIRECTION ( 'NONE',  ( 0.000000000000000000, 1.000000000000000000, -0.000000000000000000 ) ) ;
#9423=VERTEX_POINT ( 'NONE', #8850 ) ;
#9431=AXIS2_PLACEMENT_3D ( 'NONE', #2495, #9154, #9907 ) ;
#9452=DIRECTION ( 'NONE',  ( 0.9902680687415800209, 0.000000000000000000, 0.1391731009599966873 ) ) ;
#9466=FACE_BOUND ( 'NONE', #356, .T. ) ;
#9500=DIRECTION ( 'NONE',  ( 0.000000000000000000, 1.000000000000000000, -0.000000000000000000 ) ) ;
#9504=DIRECTION ( 'NONE',  ( -0.9612616959383299964, 0.000000000000000000, -0.2756373558169601945 ) ) ;
#9542=EDGE_CURVE ( 'NONE', #8191, #8559, #5078, .T. ) ;
#9551=APPLICATION_CONTEXT ( 'automotive_design' ) ;
#9652=VERTEX_POINT ( 'NONE', #10130 ) ;
#9655=AXIS2_PLACEMENT_3D ( 'NONE', #2373, #2318, #9841 ) ;
#9675=( GEOMETRIC_REPRESENTATION_CONTEXT ( 3 ) GLOBAL_UNCERTAINTY_ASSIGNED_CONTEXT ( ( #772 ) ) GLOBAL_UNIT_ASSIGNED_CONTEXT ( ( #971, #4257, #7685 ) ) REPRESENTATION_CONTEXT ( 'NONE', 'WORKASPACE' ) );
#9689=AXIS2_PLACEMENT_3D ( 'NONE', #7947, #6441, #10468 ) ;
#9690=EDGE_CURVE ( 'NONE', #9423, #10046, #2835, .T. ) ;
#9694=VECTOR ( 'NONE', #2511, 1000.000000000000000 ) ;
#9712=DIRECTION ( 'NONE',  ( 0.000000000000000000, 1.000000000000000000, -0.000000000000000000 ) ) ;
#9770=LINE ( 'NONE', #2408, #8245 ) ;
#9785=CIRCLE ( 'NONE', #2409, 4.000000000000000000 ) ;
#9841=DIRECTION ( 'NONE',  ( 0.9902680687415800209, 0.000000000000000000, 0.1391731009599966873 ) ) ;
#9844=APPLICATION_CONTEXT ( 'automotive_design' ) ;
#9868=VECTOR ( 'NONE', #9420, 1000.000000000000000 ) ;
#9903=CARTESIAN_POINT ( 'NONE',  ( -20.32733171007796713, -2.500000000000000000, -429.5091673395090766 ) ) ;
#9907=DIRECTION ( 'NONE',  ( -0.9902680687415800209, 0.000000000000000000, -0.1391731009599965763 ) ) ;
#9938=LINE ( 'NONE', #8375, #3641 ) ;
#9944=EDGE_LOOP ( 'NONE', ( #6370, #6525, #7727, #2034, #5241, #3529, #5094 ) ) ;
#9945=EDGE_CURVE ( 'NONE', #7113, #8191, #5741, .T. ) ;
#9948=AXIS2_PLACEMENT_3D ( 'NONE', #3636, #1209, #4440 ) ;
#9952=DIRECTION ( 'NONE',  ( 0.000000000000000000, 1.000000000000000000, -0.000000000000000000 ) ) ;
#9970=DIRECTION ( 'NONE',  ( -0.9612616959383299964, 0.000000000000000000, -0.2756373558169601945 ) ) ;
#9999=EDGE_CURVE ( 'NONE', #1416, #6686, #8396, .T. ) ;
#10003=SURFACE_STYLE_FILL_AREA ( #9258 ) ;
#10008=FACE_OUTER_BOUND ( 'NONE', #8289, .T. ) ;
#10046=VERTEX_POINT ( 'NONE', #3157 ) ;
#10066=CARTESIAN_POINT ( 'NONE',  ( -33.34106825788445150, -7.500000000000000000, -439.6766126514281154 ) ) ;
#10072=ORIENTED_EDGE ( 'NONE', *, *, #2264, .F. ) ;
#10073=DIRECTION ( 'NONE',  ( 0.000000000000000000, -1.000000000000000000, 0.000000000000000000 ) ) ;
#10078=DIRECTION ( 'NONE',  ( 0.000000000000000000, 1.000000000000000000, -0.000000000000000000 ) ) ;
#10117=LINE ( 'NONE', #2758, #926 ) ;
#10130=CARTESIAN_POINT ( 'NONE',  ( -45.24937426871918689, -2.500000000000000000, -448.9804009737068213 ) ) ;
#10137=AXIS2_PLACEMENT_3D ( 'NONE', #8226, #9952, #8179 ) ;
#10357=CARTESIAN_POINT ( 'NONE',  ( -28.01838671672410896, -2.500000000000000000, -497.7560445212019999 ) ) ;
#10384=DIRECTION ( 'NONE',  ( 0.000000000000000000, 1.000000000000000000, -0.000000000000000000 ) ) ;
#10423=VECTOR ( 'NONE', #7363, 1000.000000000000227 ) ;
#10453=ORIENTED_EDGE ( 'NONE', *, *, #4791, .F. ) ;
#10468=DIRECTION ( 'NONE',  ( 0.9850643254521072034, 0.000000000000000000, 0.1721867437452284377 ) ) ;
#10507=ORIENTED_EDGE ( 'NONE', *, *, #4259, .F. ) ;
#10535=EDGE_CURVE ( 'NONE', #8899, #9652, #3150, .T. ) ;
#10547=VERTEX_POINT ( 'NONE', #479 ) ;
#10550=PRODUCT_DEFINITION_CONTEXT ( 'detailed design', #9551, 'design' ) ;
#10577=CARTESIAN_POINT ( 'NONE',  ( -34.37192209820132405, -2.500000000000000000, -461.0868123482146643 ) ) ;
#10603=ORIENTED_EDGE ( 'NONE', *, *, #3484, .F. ) ;
#10618=EDGE_CURVE ( 'NONE', #7113, #10046, #4727, .T. ) ;
ENDSEC;
END-ISO-10303-21;
